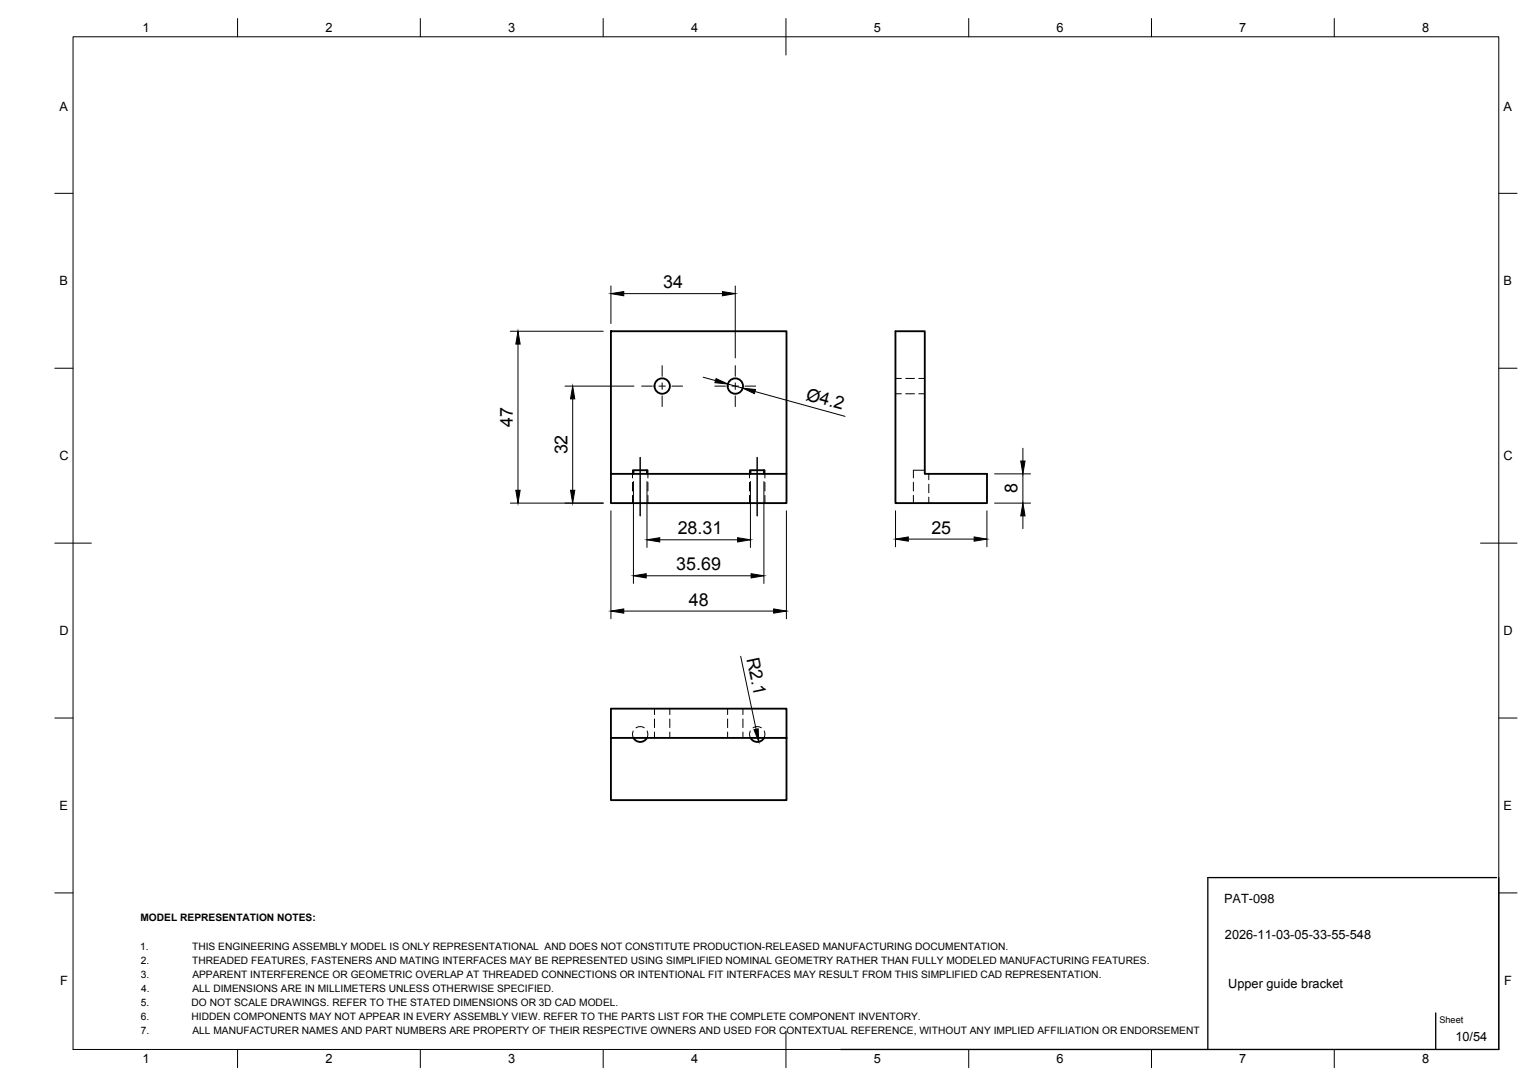
ISO-10303-21;
HEADER;
/* Generated by software containing ST-Developer
 * from STEP Tools, Inc. (www.steptools.com) 
 */

FILE_DESCRIPTION(
/* description */ ('Spring compression tester'),
/* implementation_level */ '2;1');

FILE_NAME(
/* name */ 'Upper guide bracket.step',
/* time_stamp */ '2026-10-28T03:24:11-07:00',
/* author */ (''),
/* organization */ (''),
/* preprocessor_version */ 'ST-DEVELOPER v20.2',
/* originating_system */ 'Autodesk Translation Framework v15.17.0.0',
/* authorisation */ '');

FILE_SCHEMA (('AUTOMOTIVE_DESIGN { 1 0 10303 214 3 1 1 }'));
ENDSEC;

DATA;
#10=MECHANICAL_DESIGN_GEOMETRIC_PRESENTATION_REPRESENTATION('',(#1111),#43521);
#991=SHAPE_REPRESENTATION_RELATIONSHIP('SRR','None',#43803,#1051);
#1051=ADVANCED_BREP_SHAPE_REPRESENTATION('',(#1186),#43463);
#1111=STYLED_ITEM('',(#44181),#1186);
#1186=MANIFOLD_SOLID_BREP('Body1',#18548);
#1327=FACE_BOUND('',#3415,.T.);
#1328=FACE_BOUND('',#3416,.T.);
#1329=FACE_BOUND('',#3420,.T.);
#1330=FACE_BOUND('',#3421,.T.);
#1331=FACE_BOUND('',#3424,.T.);
#1332=FACE_BOUND('',#3425,.T.);
#1653=PLANE('',#19507);
#1654=PLANE('',#19513);
#1655=PLANE('',#19514);
#1656=PLANE('',#19515);
#1657=PLANE('',#19516);
#1658=PLANE('',#19517);
#1659=PLANE('',#19518);
#1660=PLANE('',#19519);
#1661=PLANE('',#19520);
#1662=PLANE('',#19521);
#2280=FACE_OUTER_BOUND('',#3407,.T.);
#2281=FACE_OUTER_BOUND('',#3408,.T.);
#2282=FACE_OUTER_BOUND('',#3409,.T.);
#2283=FACE_OUTER_BOUND('',#3410,.T.);
#2284=FACE_OUTER_BOUND('',#3411,.T.);
#2285=FACE_OUTER_BOUND('',#3412,.T.);
#2286=FACE_OUTER_BOUND('',#3413,.T.);
#2287=FACE_OUTER_BOUND('',#3414,.T.);
#2288=FACE_OUTER_BOUND('',#3417,.T.);
#2289=FACE_OUTER_BOUND('',#3418,.T.);
#2290=FACE_OUTER_BOUND('',#3419,.T.);
#2291=FACE_OUTER_BOUND('',#3422,.T.);
#2292=FACE_OUTER_BOUND('',#3423,.T.);
#2293=FACE_OUTER_BOUND('',#3426,.T.);
#3407=EDGE_LOOP('',(#12709,#12710,#12711,#12712));
#3408=EDGE_LOOP('',(#12713,#12714,#12715,#12716));
#3409=EDGE_LOOP('',(#12717,#12718,#12719,#12720,#12721,#12722,#12723,#12724));
#3410=EDGE_LOOP('',(#12725,#12726,#12727));
#3411=EDGE_LOOP('',(#12728,#12729,#12730,#12731,#12732,#12733,#12734,#12735));
#3412=EDGE_LOOP('',(#12736,#12737,#12738));
#3413=EDGE_LOOP('',(#12739,#12740,#12741,#12742,#12743,#12744,#12745,#12746));
#3414=EDGE_LOOP('',(#12747,#12748,#12749,#12750,#12751,#12752,#12753,#12754,
#12755,#12756,#12757,#12758));
#3415=EDGE_LOOP('',(#12759));
#3416=EDGE_LOOP('',(#12760));
#3417=EDGE_LOOP('',(#12761,#12762,#12763,#12764));
#3418=EDGE_LOOP('',(#12765,#12766,#12767,#12768,#12769,#12770));
#3419=EDGE_LOOP('',(#12771,#12772,#12773,#12774));
#3420=EDGE_LOOP('',(#12775));
#3421=EDGE_LOOP('',(#12776));
#3422=EDGE_LOOP('',(#12777,#12778,#12779,#12780,#12781,#12782));
#3423=EDGE_LOOP('',(#12783,#12784,#12785,#12786));
#3424=EDGE_LOOP('',(#12787));
#3425=EDGE_LOOP('',(#12788));
#3426=EDGE_LOOP('',(#12789,#12790,#12791,#12792));
#4760=LINE('',#26986,#6192);
#4761=LINE('',#26992,#6193);
#4762=LINE('',#26998,#6194);
#4763=LINE('',#27002,#6195);
#4764=LINE('',#27006,#6196);
#4765=LINE('',#27009,#6197);
#4766=LINE('',#27014,#6198);
#4767=LINE('',#27018,#6199);
#4768=LINE('',#27022,#6200);
#4769=LINE('',#27025,#6201);
#4770=LINE('',#27027,#6202);
#4771=LINE('',#27029,#6203);
#4772=LINE('',#27031,#6204);
#4773=LINE('',#27033,#6205);
#4774=LINE('',#27035,#6206);
#4775=LINE('',#27036,#6207);
#4776=LINE('',#27039,#6208);
#4777=LINE('',#27041,#6209);
#4778=LINE('',#27042,#6210);
#4779=LINE('',#27046,#6211);
#4780=LINE('',#27047,#6212);
#4781=LINE('',#27048,#6213);
#4782=LINE('',#27052,#6214);
#4783=LINE('',#27053,#6215);
#4784=LINE('',#27054,#6216);
#4785=LINE('',#27058,#6217);
#4786=LINE('',#27059,#6218);
#4787=LINE('',#27060,#6219);
#4788=LINE('',#27062,#6220);
#4789=LINE('',#27063,#6221);
#6192=VECTOR('',#21778,0.21);
#6193=VECTOR('',#21785,0.21);
#6194=VECTOR('',#21792,0.21);
#6195=VECTOR('',#21795,1.);
#6196=VECTOR('',#21798,1.);
#6197=VECTOR('',#21803,1.);
#6198=VECTOR('',#21808,0.21);
#6199=VECTOR('',#21811,1.);
#6200=VECTOR('',#21814,1.);
#6201=VECTOR('',#21819,1.);
#6202=VECTOR('',#21822,1.);
#6203=VECTOR('',#21823,1.);
#6204=VECTOR('',#21824,1.);
#6205=VECTOR('',#21825,1.);
#6206=VECTOR('',#21826,1.);
#6207=VECTOR('',#21827,1.);
#6208=VECTOR('',#21830,1.);
#6209=VECTOR('',#21831,1.);
#6210=VECTOR('',#21832,1.);
#6211=VECTOR('',#21835,1.);
#6212=VECTOR('',#21836,1.);
#6213=VECTOR('',#21837,1.);
#6214=VECTOR('',#21840,1.);
#6215=VECTOR('',#21841,1.);
#6216=VECTOR('',#21842,1.);
#6217=VECTOR('',#21845,1.);
#6218=VECTOR('',#21846,1.);
#6219=VECTOR('',#21847,1.);
#6220=VECTOR('',#21850,1.);
#6221=VECTOR('',#21851,1.);
#7562=CIRCLE('',#19497,0.21);
#7563=CIRCLE('',#19498,0.21);
#7564=CIRCLE('',#19500,0.21);
#7565=CIRCLE('',#19501,0.21);
#7566=CIRCLE('',#19503,0.21);
#7567=CIRCLE('',#19504,0.21);
#7568=CIRCLE('',#19505,0.21);
#7569=CIRCLE('',#19506,0.21);
#7570=CIRCLE('',#19509,0.21);
#7571=CIRCLE('',#19510,0.21);
#7572=CIRCLE('',#19511,0.21);
#7573=CIRCLE('',#19512,0.21);
#8300=VERTEX_POINT('',#26983);
#8301=VERTEX_POINT('',#26985);
#8302=VERTEX_POINT('',#26989);
#8303=VERTEX_POINT('',#26991);
#8304=VERTEX_POINT('',#26995);
#8305=VERTEX_POINT('',#26997);
#8306=VERTEX_POINT('',#26999);
#8307=VERTEX_POINT('',#27001);
#8308=VERTEX_POINT('',#27003);
#8309=VERTEX_POINT('',#27005);
#8310=VERTEX_POINT('',#27011);
#8311=VERTEX_POINT('',#27013);
#8312=VERTEX_POINT('',#27015);
#8313=VERTEX_POINT('',#27017);
#8314=VERTEX_POINT('',#27019);
#8315=VERTEX_POINT('',#27021);
#8316=VERTEX_POINT('',#27028);
#8317=VERTEX_POINT('',#27030);
#8318=VERTEX_POINT('',#27032);
#8319=VERTEX_POINT('',#27034);
#8320=VERTEX_POINT('',#27038);
#8321=VERTEX_POINT('',#27040);
#8322=VERTEX_POINT('',#27044);
#8323=VERTEX_POINT('',#27045);
#8324=VERTEX_POINT('',#27050);
#8325=VERTEX_POINT('',#27051);
#8326=VERTEX_POINT('',#27056);
#8327=VERTEX_POINT('',#27057);
#10019=EDGE_CURVE('',#8300,#8300,#7562,.T.);
#10020=EDGE_CURVE('',#8300,#8301,#4760,.T.);
#10021=EDGE_CURVE('',#8301,#8301,#7563,.T.);
#10022=EDGE_CURVE('',#8302,#8302,#7564,.T.);
#10023=EDGE_CURVE('',#8302,#8303,#4761,.T.);
#10024=EDGE_CURVE('',#8303,#8303,#7565,.T.);
#10025=EDGE_CURVE('',#8304,#8304,#7566,.T.);
#10026=EDGE_CURVE('',#8304,#8305,#4762,.T.);
#10027=EDGE_CURVE('',#8305,#8306,#7567,.T.);
#10028=EDGE_CURVE('',#8307,#8306,#4763,.T.);
#10029=EDGE_CURVE('',#8308,#8307,#7568,.T.);
#10030=EDGE_CURVE('',#8309,#8308,#4764,.T.);
#10031=EDGE_CURVE('',#8309,#8305,#7569,.T.);
#10032=EDGE_CURVE('',#8306,#8309,#4765,.T.);
#10033=EDGE_CURVE('',#8310,#8310,#7570,.T.);
#10034=EDGE_CURVE('',#8310,#8311,#4766,.T.);
#10035=EDGE_CURVE('',#8311,#8312,#7571,.T.);
#10036=EDGE_CURVE('',#8313,#8312,#4767,.T.);
#10037=EDGE_CURVE('',#8314,#8313,#7572,.T.);
#10038=EDGE_CURVE('',#8315,#8314,#4768,.T.);
#10039=EDGE_CURVE('',#8315,#8311,#7573,.T.);
#10040=EDGE_CURVE('',#8312,#8315,#4769,.T.);
#10041=EDGE_CURVE('',#8307,#8314,#4770,.T.);
#10042=EDGE_CURVE('',#8313,#8316,#4771,.T.);
#10043=EDGE_CURVE('',#8317,#8316,#4772,.T.);
#10044=EDGE_CURVE('',#8317,#8318,#4773,.T.);
#10045=EDGE_CURVE('',#8318,#8319,#4774,.T.);
#10046=EDGE_CURVE('',#8319,#8308,#4775,.T.);
#10047=EDGE_CURVE('',#8319,#8320,#4776,.T.);
#10048=EDGE_CURVE('',#8321,#8320,#4777,.T.);
#10049=EDGE_CURVE('',#8316,#8321,#4778,.T.);
#10050=EDGE_CURVE('',#8322,#8323,#4779,.T.);
#10051=EDGE_CURVE('',#8323,#8321,#4780,.T.);
#10052=EDGE_CURVE('',#8320,#8322,#4781,.T.);
#10053=EDGE_CURVE('',#8324,#8325,#4782,.T.);
#10054=EDGE_CURVE('',#8324,#8317,#4783,.T.);
#10055=EDGE_CURVE('',#8325,#8323,#4784,.T.);
#10056=EDGE_CURVE('',#8326,#8327,#4785,.T.);
#10057=EDGE_CURVE('',#8326,#8324,#4786,.T.);
#10058=EDGE_CURVE('',#8327,#8325,#4787,.T.);
#10059=EDGE_CURVE('',#8318,#8326,#4788,.T.);
#10060=EDGE_CURVE('',#8327,#8322,#4789,.T.);
#12709=ORIENTED_EDGE('',*,*,#10019,.F.);
#12710=ORIENTED_EDGE('',*,*,#10020,.T.);
#12711=ORIENTED_EDGE('',*,*,#10021,.F.);
#12712=ORIENTED_EDGE('',*,*,#10020,.F.);
#12713=ORIENTED_EDGE('',*,*,#10022,.F.);
#12714=ORIENTED_EDGE('',*,*,#10023,.T.);
#12715=ORIENTED_EDGE('',*,*,#10024,.F.);
#12716=ORIENTED_EDGE('',*,*,#10023,.F.);
#12717=ORIENTED_EDGE('',*,*,#10025,.F.);
#12718=ORIENTED_EDGE('',*,*,#10026,.T.);
#12719=ORIENTED_EDGE('',*,*,#10027,.T.);
#12720=ORIENTED_EDGE('',*,*,#10028,.F.);
#12721=ORIENTED_EDGE('',*,*,#10029,.F.);
#12722=ORIENTED_EDGE('',*,*,#10030,.F.);
#12723=ORIENTED_EDGE('',*,*,#10031,.T.);
#12724=ORIENTED_EDGE('',*,*,#10026,.F.);
#12725=ORIENTED_EDGE('',*,*,#10032,.F.);
#12726=ORIENTED_EDGE('',*,*,#10027,.F.);
#12727=ORIENTED_EDGE('',*,*,#10031,.F.);
#12728=ORIENTED_EDGE('',*,*,#10033,.F.);
#12729=ORIENTED_EDGE('',*,*,#10034,.T.);
#12730=ORIENTED_EDGE('',*,*,#10035,.T.);
#12731=ORIENTED_EDGE('',*,*,#10036,.F.);
#12732=ORIENTED_EDGE('',*,*,#10037,.F.);
#12733=ORIENTED_EDGE('',*,*,#10038,.F.);
#12734=ORIENTED_EDGE('',*,*,#10039,.T.);
#12735=ORIENTED_EDGE('',*,*,#10034,.F.);
#12736=ORIENTED_EDGE('',*,*,#10040,.F.);
#12737=ORIENTED_EDGE('',*,*,#10035,.F.);
#12738=ORIENTED_EDGE('',*,*,#10039,.F.);
#12739=ORIENTED_EDGE('',*,*,#10029,.T.);
#12740=ORIENTED_EDGE('',*,*,#10041,.T.);
#12741=ORIENTED_EDGE('',*,*,#10037,.T.);
#12742=ORIENTED_EDGE('',*,*,#10042,.T.);
#12743=ORIENTED_EDGE('',*,*,#10043,.F.);
#12744=ORIENTED_EDGE('',*,*,#10044,.T.);
#12745=ORIENTED_EDGE('',*,*,#10045,.T.);
#12746=ORIENTED_EDGE('',*,*,#10046,.T.);
#12747=ORIENTED_EDGE('',*,*,#10030,.T.);
#12748=ORIENTED_EDGE('',*,*,#10046,.F.);
#12749=ORIENTED_EDGE('',*,*,#10047,.T.);
#12750=ORIENTED_EDGE('',*,*,#10048,.F.);
#12751=ORIENTED_EDGE('',*,*,#10049,.F.);
#12752=ORIENTED_EDGE('',*,*,#10042,.F.);
#12753=ORIENTED_EDGE('',*,*,#10036,.T.);
#12754=ORIENTED_EDGE('',*,*,#10040,.T.);
#12755=ORIENTED_EDGE('',*,*,#10038,.T.);
#12756=ORIENTED_EDGE('',*,*,#10041,.F.);
#12757=ORIENTED_EDGE('',*,*,#10028,.T.);
#12758=ORIENTED_EDGE('',*,*,#10032,.T.);
#12759=ORIENTED_EDGE('',*,*,#10019,.T.);
#12760=ORIENTED_EDGE('',*,*,#10022,.T.);
#12761=ORIENTED_EDGE('',*,*,#10050,.T.);
#12762=ORIENTED_EDGE('',*,*,#10051,.T.);
#12763=ORIENTED_EDGE('',*,*,#10048,.T.);
#12764=ORIENTED_EDGE('',*,*,#10052,.T.);
#12765=ORIENTED_EDGE('',*,*,#10053,.F.);
#12766=ORIENTED_EDGE('',*,*,#10054,.T.);
#12767=ORIENTED_EDGE('',*,*,#10043,.T.);
#12768=ORIENTED_EDGE('',*,*,#10049,.T.);
#12769=ORIENTED_EDGE('',*,*,#10051,.F.);
#12770=ORIENTED_EDGE('',*,*,#10055,.F.);
#12771=ORIENTED_EDGE('',*,*,#10056,.F.);
#12772=ORIENTED_EDGE('',*,*,#10057,.T.);
#12773=ORIENTED_EDGE('',*,*,#10053,.T.);
#12774=ORIENTED_EDGE('',*,*,#10058,.F.);
#12775=ORIENTED_EDGE('',*,*,#10025,.T.);
#12776=ORIENTED_EDGE('',*,*,#10033,.T.);
#12777=ORIENTED_EDGE('',*,*,#10045,.F.);
#12778=ORIENTED_EDGE('',*,*,#10059,.T.);
#12779=ORIENTED_EDGE('',*,*,#10056,.T.);
#12780=ORIENTED_EDGE('',*,*,#10060,.T.);
#12781=ORIENTED_EDGE('',*,*,#10052,.F.);
#12782=ORIENTED_EDGE('',*,*,#10047,.F.);
#12783=ORIENTED_EDGE('',*,*,#10060,.F.);
#12784=ORIENTED_EDGE('',*,*,#10058,.T.);
#12785=ORIENTED_EDGE('',*,*,#10055,.T.);
#12786=ORIENTED_EDGE('',*,*,#10050,.F.);
#12787=ORIENTED_EDGE('',*,*,#10021,.T.);
#12788=ORIENTED_EDGE('',*,*,#10024,.T.);
#12789=ORIENTED_EDGE('',*,*,#10059,.F.);
#12790=ORIENTED_EDGE('',*,*,#10044,.F.);
#12791=ORIENTED_EDGE('',*,*,#10054,.F.);
#12792=ORIENTED_EDGE('',*,*,#10057,.F.);
#17151=CYLINDRICAL_SURFACE('',#19496,0.21);
#17152=CYLINDRICAL_SURFACE('',#19499,0.21);
#17153=CYLINDRICAL_SURFACE('',#19502,0.21);
#17154=CYLINDRICAL_SURFACE('',#19508,0.21);
#17604=ADVANCED_FACE('',(#2280),#17151,.F.);
#17605=ADVANCED_FACE('',(#2281),#17152,.F.);
#17606=ADVANCED_FACE('',(#2282),#17153,.F.);
#17607=ADVANCED_FACE('',(#2283),#1653,.F.);
#17608=ADVANCED_FACE('',(#2284),#17154,.F.);
#17609=ADVANCED_FACE('',(#2285),#1654,.F.);
#17610=ADVANCED_FACE('',(#2286),#1655,.T.);
#17611=ADVANCED_FACE('',(#2287,#1327,#1328),#1656,.T.);
#17612=ADVANCED_FACE('',(#2288),#1657,.T.);
#17613=ADVANCED_FACE('',(#2289),#1658,.T.);
#17614=ADVANCED_FACE('',(#2290,#1329,#1330),#1659,.T.);
#17615=ADVANCED_FACE('',(#2291),#1660,.T.);
#17616=ADVANCED_FACE('',(#2292,#1331,#1332),#1661,.T.);
#17617=ADVANCED_FACE('',(#2293),#1662,.F.);
#18548=CLOSED_SHELL('',(#17604,#17605,#17606,#17607,#17608,#17609,#17610,
#17611,#17612,#17613,#17614,#17615,#17616,#17617));
#19495=AXIS2_PLACEMENT_3D('',#26981,#21772,#21773);
#19496=AXIS2_PLACEMENT_3D('',#26982,#21774,#21775);
#19497=AXIS2_PLACEMENT_3D('',#26984,#21776,#21777);
#19498=AXIS2_PLACEMENT_3D('',#26987,#21779,#21780);
#19499=AXIS2_PLACEMENT_3D('',#26988,#21781,#21782);
#19500=AXIS2_PLACEMENT_3D('',#26990,#21783,#21784);
#19501=AXIS2_PLACEMENT_3D('',#26993,#21786,#21787);
#19502=AXIS2_PLACEMENT_3D('',#26994,#21788,#21789);
#19503=AXIS2_PLACEMENT_3D('',#26996,#21790,#21791);
#19504=AXIS2_PLACEMENT_3D('',#27000,#21793,#21794);
#19505=AXIS2_PLACEMENT_3D('',#27004,#21796,#21797);
#19506=AXIS2_PLACEMENT_3D('',#27007,#21799,#21800);
#19507=AXIS2_PLACEMENT_3D('',#27008,#21801,#21802);
#19508=AXIS2_PLACEMENT_3D('',#27010,#21804,#21805);
#19509=AXIS2_PLACEMENT_3D('',#27012,#21806,#21807);
#19510=AXIS2_PLACEMENT_3D('',#27016,#21809,#21810);
#19511=AXIS2_PLACEMENT_3D('',#27020,#21812,#21813);
#19512=AXIS2_PLACEMENT_3D('',#27023,#21815,#21816);
#19513=AXIS2_PLACEMENT_3D('',#27024,#21817,#21818);
#19514=AXIS2_PLACEMENT_3D('',#27026,#21820,#21821);
#19515=AXIS2_PLACEMENT_3D('',#27037,#21828,#21829);
#19516=AXIS2_PLACEMENT_3D('',#27043,#21833,#21834);
#19517=AXIS2_PLACEMENT_3D('',#27049,#21838,#21839);
#19518=AXIS2_PLACEMENT_3D('',#27055,#21843,#21844);
#19519=AXIS2_PLACEMENT_3D('',#27061,#21848,#21849);
#19520=AXIS2_PLACEMENT_3D('',#27064,#21852,#21853);
#19521=AXIS2_PLACEMENT_3D('',#27065,#21854,#21855);
#21772=DIRECTION('axis',(0.,0.,1.));
#21773=DIRECTION('refdir',(1.,0.,0.));
#21774=DIRECTION('center_axis',(0.,0.,1.));
#21775=DIRECTION('ref_axis',(1.,0.,0.));
#21776=DIRECTION('center_axis',(0.,0.,1.));
#21777=DIRECTION('ref_axis',(1.,0.,0.));
#21778=DIRECTION('',(0.,0.,1.));
#21779=DIRECTION('center_axis',(0.,0.,-1.));
#21780=DIRECTION('ref_axis',(1.,0.,0.));
#21781=DIRECTION('center_axis',(0.,0.,1.));
#21782=DIRECTION('ref_axis',(1.,0.,0.));
#21783=DIRECTION('center_axis',(0.,0.,1.));
#21784=DIRECTION('ref_axis',(1.,0.,0.));
#21785=DIRECTION('',(0.,0.,1.));
#21786=DIRECTION('center_axis',(0.,0.,-1.));
#21787=DIRECTION('ref_axis',(1.,0.,0.));
#21788=DIRECTION('center_axis',(0.,1.,0.));
#21789=DIRECTION('ref_axis',(1.,0.,0.));
#21790=DIRECTION('center_axis',(0.,1.,0.));
#21791=DIRECTION('ref_axis',(1.,0.,0.));
#21792=DIRECTION('',(0.,1.,0.));
#21793=DIRECTION('center_axis',(0.,1.,0.));
#21794=DIRECTION('ref_axis',(1.,0.,0.));
#21795=DIRECTION('',(0.,1.,0.));
#21796=DIRECTION('center_axis',(0.,-1.,0.));
#21797=DIRECTION('ref_axis',(1.,0.,0.));
#21798=DIRECTION('',(0.,-1.,0.));
#21799=DIRECTION('center_axis',(0.,1.,0.));
#21800=DIRECTION('ref_axis',(1.,0.,0.));
#21801=DIRECTION('center_axis',(0.,1.,0.));
#21802=DIRECTION('ref_axis',(1.,0.,0.));
#21803=DIRECTION('',(-1.,0.,0.));
#21804=DIRECTION('center_axis',(0.,1.,0.));
#21805=DIRECTION('ref_axis',(1.,0.,0.));
#21806=DIRECTION('center_axis',(0.,1.,0.));
#21807=DIRECTION('ref_axis',(1.,0.,0.));
#21808=DIRECTION('',(0.,1.,0.));
#21809=DIRECTION('center_axis',(0.,1.,0.));
#21810=DIRECTION('ref_axis',(1.,0.,0.));
#21811=DIRECTION('',(0.,1.,0.));
#21812=DIRECTION('center_axis',(0.,-1.,0.));
#21813=DIRECTION('ref_axis',(1.,0.,0.));
#21814=DIRECTION('',(0.,-1.,0.));
#21815=DIRECTION('center_axis',(0.,1.,0.));
#21816=DIRECTION('ref_axis',(1.,0.,0.));
#21817=DIRECTION('center_axis',(0.,1.,0.));
#21818=DIRECTION('ref_axis',(1.,0.,0.));
#21819=DIRECTION('',(-1.,0.,0.));
#21820=DIRECTION('center_axis',(0.,1.,0.));
#21821=DIRECTION('ref_axis',(-1.,0.,0.));
#21822=DIRECTION('',(1.,0.,0.));
#21823=DIRECTION('',(1.,0.,0.));
#21824=DIRECTION('',(0.,0.,1.));
#21825=DIRECTION('',(-1.,0.,0.));
#21826=DIRECTION('',(0.,0.,1.));
#21827=DIRECTION('',(1.,0.,0.));
#21828=DIRECTION('center_axis',(0.,0.,-1.));
#21829=DIRECTION('ref_axis',(-1.,0.,0.));
#21830=DIRECTION('',(0.,1.,0.));
#21831=DIRECTION('',(-1.,0.,0.));
#21832=DIRECTION('',(0.,1.,0.));
#21833=DIRECTION('center_axis',(0.,1.,0.));
#21834=DIRECTION('ref_axis',(0.,0.,1.));
#21835=DIRECTION('',(1.,0.,0.));
#21836=DIRECTION('',(0.,0.,-1.));
#21837=DIRECTION('',(0.,0.,1.));
#21838=DIRECTION('center_axis',(1.,0.,0.));
#21839=DIRECTION('ref_axis',(0.,1.,0.));
#21840=DIRECTION('',(0.,0.,1.));
#21841=DIRECTION('',(0.,1.,0.));
#21842=DIRECTION('',(0.,1.,0.));
#21843=DIRECTION('center_axis',(0.,-1.,0.));
#21844=DIRECTION('ref_axis',(1.,0.,0.));
#21845=DIRECTION('',(0.,0.,1.));
#21846=DIRECTION('',(1.,0.,0.));
#21847=DIRECTION('',(1.,0.,0.));
#21848=DIRECTION('center_axis',(-1.,0.,0.));
#21849=DIRECTION('ref_axis',(0.,-1.,0.));
#21850=DIRECTION('',(0.,-1.,0.));
#21851=DIRECTION('',(0.,1.,0.));
#21852=DIRECTION('center_axis',(0.,0.,1.));
#21853=DIRECTION('ref_axis',(1.,0.,0.));
#21854=DIRECTION('center_axis',(0.,0.,1.));
#21855=DIRECTION('ref_axis',(1.,0.,0.));
#26981=CARTESIAN_POINT('',(0.,0.,0.));
#26982=CARTESIAN_POINT('Origin',(-7.,5.5,29.6));
#26983=CARTESIAN_POINT('',(-7.21,5.5,29.7));
#26984=CARTESIAN_POINT('Origin',(-7.,5.5,29.7));
#26985=CARTESIAN_POINT('',(-7.21,5.5,30.5));
#26986=CARTESIAN_POINT('',(-7.21,5.5,29.6));
#26987=CARTESIAN_POINT('Origin',(-7.,5.5,30.5));
#26988=CARTESIAN_POINT('Origin',(-5.,5.5,29.6));
#26989=CARTESIAN_POINT('',(-5.21,5.5,29.7));
#26990=CARTESIAN_POINT('Origin',(-5.,5.5,29.7));
#26991=CARTESIAN_POINT('',(-5.21,5.5,30.5));
#26992=CARTESIAN_POINT('',(-5.21,5.5,29.6));
#26993=CARTESIAN_POINT('Origin',(-5.,5.5,30.5));
#26994=CARTESIAN_POINT('Origin',(-7.6,2.2,29.8));
#26995=CARTESIAN_POINT('',(-7.81,2.3,29.8));
#26996=CARTESIAN_POINT('Origin',(-7.6,2.3,29.8));
#26997=CARTESIAN_POINT('',(-7.81,3.2,29.8));
#26998=CARTESIAN_POINT('',(-7.81,2.2,29.8));
#26999=CARTESIAN_POINT('',(-7.41533814687381,3.2,29.7));
#27000=CARTESIAN_POINT('Origin',(-7.6,3.2,29.8));
#27001=CARTESIAN_POINT('',(-7.4153381468738,3.1,29.7));
#27002=CARTESIAN_POINT('',(-7.41533814687381,2.2,29.7));
#27003=CARTESIAN_POINT('',(-7.78466185312619,3.1,29.7));
#27004=CARTESIAN_POINT('Origin',(-7.6,3.1,29.8));
#27005=CARTESIAN_POINT('',(-7.78466185312619,3.2,29.7));
#27006=CARTESIAN_POINT('',(-7.78466185312619,2.2,29.7));
#27007=CARTESIAN_POINT('Origin',(-7.6,3.2,29.8));
#27008=CARTESIAN_POINT('Origin',(-7.6,3.2,29.8));
#27009=CARTESIAN_POINT('',(-5.6,3.2,29.7));
#27010=CARTESIAN_POINT('Origin',(-4.4,2.2,29.8));
#27011=CARTESIAN_POINT('',(-4.61,2.3,29.8));
#27012=CARTESIAN_POINT('Origin',(-4.4,2.3,29.8));
#27013=CARTESIAN_POINT('',(-4.61,3.2,29.8));
#27014=CARTESIAN_POINT('',(-4.61,2.2,29.8));
#27015=CARTESIAN_POINT('',(-4.21533814687381,3.2,29.7));
#27016=CARTESIAN_POINT('Origin',(-4.4,3.2,29.8));
#27017=CARTESIAN_POINT('',(-4.21533814687381,3.1,29.7));
#27018=CARTESIAN_POINT('',(-4.21533814687381,2.2,29.7));
#27019=CARTESIAN_POINT('',(-4.5846618531262,3.1,29.7));
#27020=CARTESIAN_POINT('Origin',(-4.4,3.1,29.8));
#27021=CARTESIAN_POINT('',(-4.58466185312619,3.2,29.7));
#27022=CARTESIAN_POINT('',(-4.58466185312619,2.2,29.7));
#27023=CARTESIAN_POINT('Origin',(-4.4,3.2,29.8));
#27024=CARTESIAN_POINT('Origin',(-4.4,3.2,29.8));
#27025=CARTESIAN_POINT('',(-4.,3.2,29.7));
#27026=CARTESIAN_POINT('Origin',(-3.6,3.1,28.));
#27027=CARTESIAN_POINT('',(-3.6,3.1,29.7));
#27028=CARTESIAN_POINT('',(-3.6,3.1,29.7));
#27029=CARTESIAN_POINT('',(-3.6,3.1,29.7));
#27030=CARTESIAN_POINT('',(-3.6,3.1,28.));
#27031=CARTESIAN_POINT('',(-3.6,3.1,28.));
#27032=CARTESIAN_POINT('',(-8.4,3.1,28.));
#27033=CARTESIAN_POINT('',(-3.6,3.1,28.));
#27034=CARTESIAN_POINT('',(-8.4,3.1,29.7));
#27035=CARTESIAN_POINT('',(-8.4,3.1,28.));
#27036=CARTESIAN_POINT('',(-3.6,3.1,29.7));
#27037=CARTESIAN_POINT('Origin',(-3.6,2.3,29.7));
#27038=CARTESIAN_POINT('',(-8.4,7.,29.7));
#27039=CARTESIAN_POINT('',(-8.4,2.3,29.7));
#27040=CARTESIAN_POINT('',(-3.6,7.,29.7));
#27041=CARTESIAN_POINT('',(-8.4,7.,29.7));
#27042=CARTESIAN_POINT('',(-3.6,2.3,29.7));
#27043=CARTESIAN_POINT('Origin',(-6.,7.,30.1));
#27044=CARTESIAN_POINT('',(-8.4,7.,30.5));
#27045=CARTESIAN_POINT('',(-3.6,7.,30.5));
#27046=CARTESIAN_POINT('',(-3.6,7.,30.5));
#27047=CARTESIAN_POINT('',(-3.6,7.,29.7));
#27048=CARTESIAN_POINT('',(-8.4,7.,30.5));
#27049=CARTESIAN_POINT('Origin',(-3.6,2.3,28.));
#27050=CARTESIAN_POINT('',(-3.6,2.3,28.));
#27051=CARTESIAN_POINT('',(-3.6,2.3,30.5));
#27052=CARTESIAN_POINT('',(-3.6,2.3,28.));
#27053=CARTESIAN_POINT('',(-3.6,2.3,28.));
#27054=CARTESIAN_POINT('',(-3.6,2.3,30.5));
#27055=CARTESIAN_POINT('Origin',(-8.4,2.3,28.));
#27056=CARTESIAN_POINT('',(-8.4,2.3,28.));
#27057=CARTESIAN_POINT('',(-8.4,2.3,30.5));
#27058=CARTESIAN_POINT('',(-8.4,2.3,28.));
#27059=CARTESIAN_POINT('',(-8.4,2.3,28.));
#27060=CARTESIAN_POINT('',(-8.4,2.3,30.5));
#27061=CARTESIAN_POINT('Origin',(-8.4,3.1,28.));
#27062=CARTESIAN_POINT('',(-8.4,3.1,28.));
#27063=CARTESIAN_POINT('',(-8.4,2.3,30.5));
#27064=CARTESIAN_POINT('Origin',(-6.,2.7,30.5));
#27065=CARTESIAN_POINT('Origin',(-6.,2.7,28.));
#43395=UNCERTAINTY_MEASURE_WITH_UNIT(LENGTH_MEASURE(0.001),#43522,
'DISTANCE_ACCURACY_VALUE',
'Maximum model space distance between geometric entities at asserted c
onnectivities');
#43453=UNCERTAINTY_MEASURE_WITH_UNIT(LENGTH_MEASURE(0.001),#43522,
'DISTANCE_ACCURACY_VALUE',
'Maximum model space distance between geometric entities at asserted c
onnectivities');
#43463=(
GEOMETRIC_REPRESENTATION_CONTEXT(3)
GLOBAL_UNCERTAINTY_ASSIGNED_CONTEXT((#43395))
GLOBAL_UNIT_ASSIGNED_CONTEXT((#43522,#43524,#43525))
REPRESENTATION_CONTEXT('','3D')
);
#43521=(
GEOMETRIC_REPRESENTATION_CONTEXT(3)
GLOBAL_UNCERTAINTY_ASSIGNED_CONTEXT((#43453))
GLOBAL_UNIT_ASSIGNED_CONTEXT((#43522,#43524,#43525))
REPRESENTATION_CONTEXT('','3D')
);
#43522=(
LENGTH_UNIT()
NAMED_UNIT(*)
SI_UNIT(.CENTI.,.METRE.)
);
#43524=(
NAMED_UNIT(*)
PLANE_ANGLE_UNIT()
SI_UNIT($,.RADIAN.)
);
#43525=(
NAMED_UNIT(*)
SI_UNIT($,.STERADIAN.)
SOLID_ANGLE_UNIT()
);
#43535=SHAPE_DEFINITION_REPRESENTATION(#43602,#43803);
#43602=PRODUCT_DEFINITION_SHAPE('',$,#43871);
#43803=SHAPE_REPRESENTATION('',(#19495),#43463);
#43861=PRODUCT_DEFINITION_CONTEXT('part definition',#44064,'design');
#43871=PRODUCT_DEFINITION('Upper guide bracket','Upper guide bracket',#43938,
#43861);
#43938=PRODUCT_DEFINITION_FORMATION('',$,#44075);
#44064=APPLICATION_CONTEXT(
'Core Data for Automotive Mechanical Design Process');
#44065=PRODUCT_CONTEXT('part definition',#44064,'mechanical');
#44075=PRODUCT('Upper guide bracket','Upper guide bracket',
'Upper guide bracket',(#44065));
#44175=COLOUR_RGB('Dark Blue',0.08,0.2,0.34);
#44176=FILL_AREA_STYLE_COLOUR('',#44175);
#44177=FILL_AREA_STYLE('',(#44176));
#44178=SURFACE_STYLE_FILL_AREA(#44177);
#44179=SURFACE_SIDE_STYLE('',(#44178));
#44180=SURFACE_STYLE_USAGE(.BOTH.,#44179);
#44181=PRESENTATION_STYLE_ASSIGNMENT((#44180));
ENDSEC;
END-ISO-10303-21;
